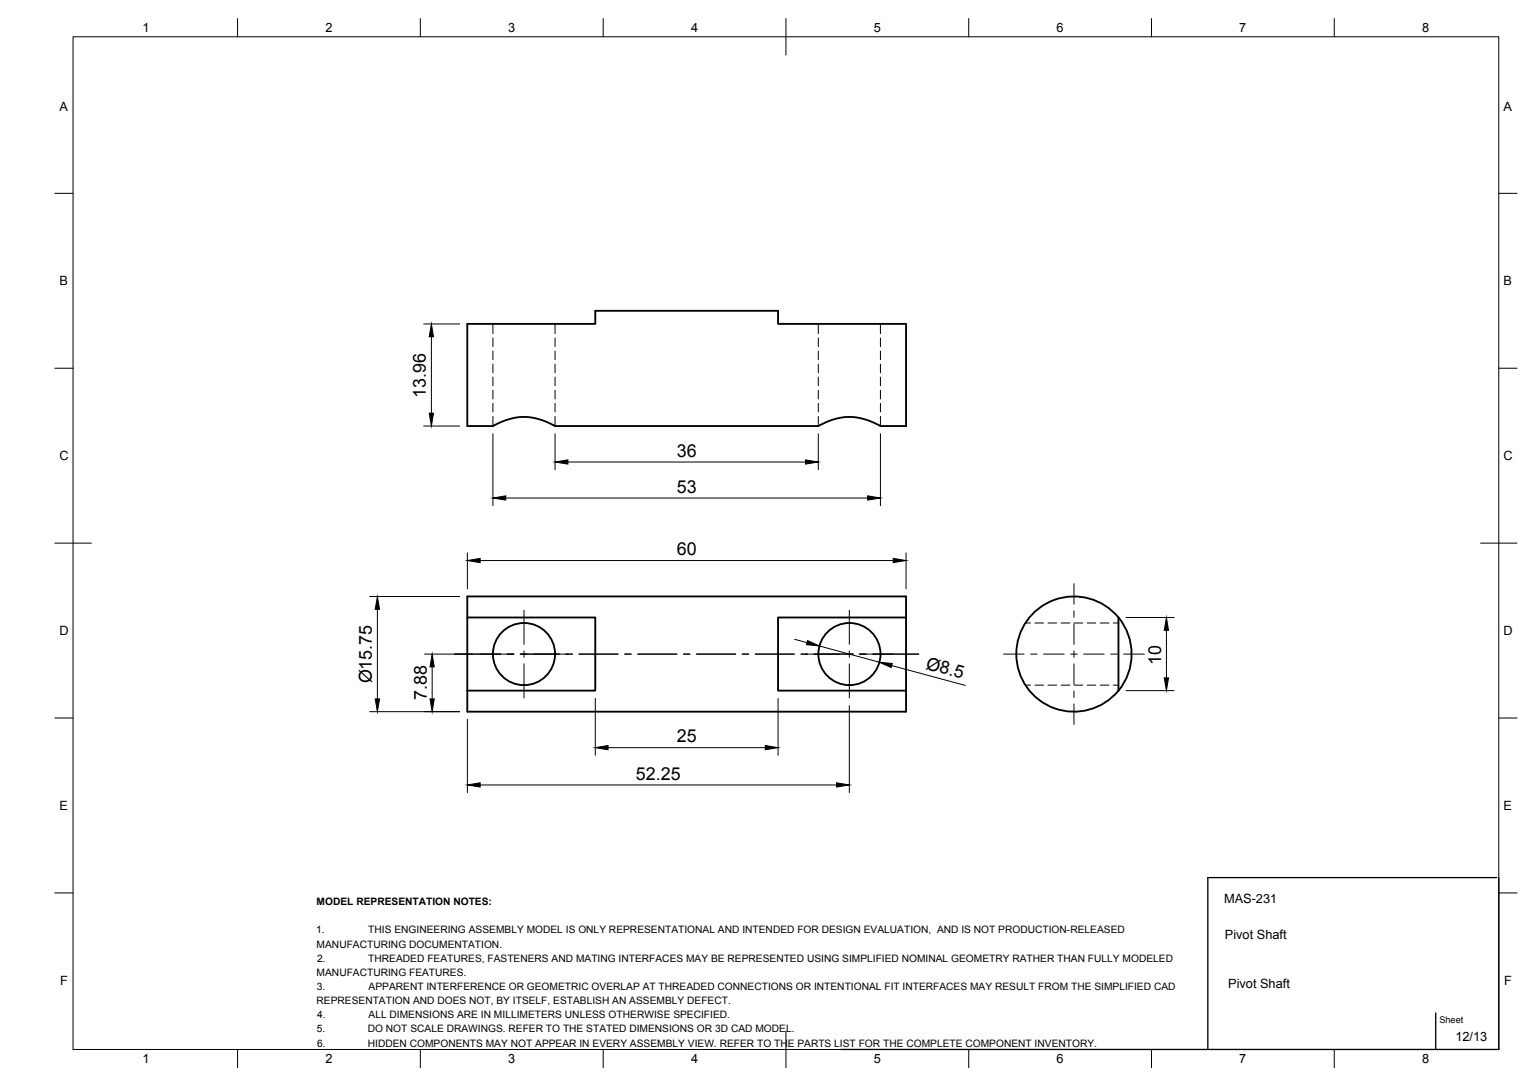
ISO-10303-21;
HEADER;
FILE_DESCRIPTION (('STEP AP214'),
    '1' );
FILE_NAME ( 'Pivot Shaft.step', '2026-10-04T02:08:54', ( '' ), ( '' ), 'STEP AP214', 'Unspecified', '' );
FILE_SCHEMA (( 'AUTOMOTIVE_DESIGN' ));
ENDSEC;
DATA;
#94=LINE ( 'NONE', #8474, #24641 ) ;
#163=CARTESIAN_POINT ( 'NONE',  ( 0.000000000000000000, 0.000000000000000000, 1.181102362204724310 ) ) ;
#167=FACE_BOUND ( 'NONE', #12224, .T. ) ;
#448=CARTESIAN_POINT ( 'NONE',  ( -0.3100393700787401619, -2.714815113292586694E-26, 1.043307086614172707 ) ) ;
#641=CARTESIAN_POINT ( 'NONE',  ( -0.3094175599200251203, 0.02245875686878780197, -0.7098059324661201153 ) ) ;
#676=CARTESIAN_POINT ( 'NONE',  ( -0.2802144182493691016, 0.1328525842424023995, 0.9782784368059546098 ) ) ;
#685=CARTESIAN_POINT ( 'NONE',  ( 0.2395294000716133853, 0.1968503937007874127, -1.181102362204724310 ) ) ;
#708=B_SPLINE_CURVE_WITH_KNOTS ( 'NONE', 3,
 ( #28141, #32202, #2466, #28627, #9914, #21640, #28865, #17093, #7013, #18040, #32685, #28374, #6538, #32454, #24524, #2926, #25235, #7260, #47275, #6296, #31966, #42943, #39824, #46788, #14454, #29112, #43665, #35327, #13976, #46551, #21152, #25494, #20919, #10153, #47031, #17804, #35559, #10873 ),
 .UNSPECIFIED., .F., .F.,
 ( 4, 2, 2, 2, 2, 2, 2, 2, 2, 2, 2, 2, 2, 2, 2, 2, 2, 2, 4 ),
 ( 0.000000000000000000, 0.0008476847199669468704, 0.001695369439933893741, 0.002543054159900840286, 0.003390738879867787482, 0.004238423599834733810, 0.005086108319801680572, 0.005933793039768628201, 0.006781477759735574963, 0.007205320119719049211, 0.007629162479702521725, 0.008476847199669457211, 0.009324531919636393565, 0.01017221663960332992, 0.01101990135957026627, 0.01186758607953720263, 0.01229142843952067167, 0.01271527079950414071, 0.01356295551947107707 ),
 .UNSPECIFIED. ) ;
#738=ADVANCED_FACE ( 'NONE', ( #36391 ), #37067, .F. ) ;
#834=VECTOR ( 'NONE', #5877, 39.37007874015748143 ) ;
#862=CARTESIAN_POINT ( 'NONE',  ( 0.2395294000716133853, 0.000000000000000000, 0.8759842519685039353 ) ) ;
#983=ORIENTED_EDGE ( 'NONE', *, *, #25046, .T. ) ;
#1196=AXIS2_PLACEMENT_3D ( 'NONE', #37509, #40374, #15249 ) ;
#1391=ORIENTED_EDGE ( 'NONE', *, *, #22168, .T. ) ;
#1402=DIRECTION ( 'NONE',  ( -1.000000000000000000, 0.000000000000000000, 0.000000000000000000 ) ) ;
#1442=CARTESIAN_POINT ( 'NONE',  ( -0.3100393700787401619, -2.714815113292586694E-26, 1.043307086614172707 ) ) ;
#1445=ADVANCED_FACE ( 'NONE', ( #167, #29705 ), #40878, .F. ) ;
#1497=CARTESIAN_POINT ( 'NONE',  ( 0.000000000000000000, 0.000000000000000000, -0.4921259842519685179 ) ) ;
#1651=VERTEX_POINT ( 'NONE', #38262 ) ;
#1728=CARTESIAN_POINT ( 'NONE',  ( -0.2984771744461587883, -0.08441368980803264088, 1.020863600671442217 ) ) ;
#1893=VERTEX_POINT ( 'NONE', #8023 ) ;
#2183=LINE ( 'NONE', #28090, #23824 ) ;
#2229=CARTESIAN_POINT ( 'NONE',  ( 0.2395294000716134131, 3.423225304703229610E-16, -0.7086614173228350522 ) ) ;
#2328=VERTEX_POINT ( 'NONE', #25156 ) ;
#2358=AXIS2_PLACEMENT_3D ( 'NONE', #3227, #47084, #17858 ) ;
#2433=EDGE_CURVE ( 'NONE', #33511, #19692, #3856, .T. ) ;
#2466=CARTESIAN_POINT ( 'NONE',  ( -0.3094241246319156535, -0.02236840013889242890, -1.042174736855756789 ) ) ;
#2926=CARTESIAN_POINT ( 'NONE',  ( -0.2617501178043720178, -0.1661865978653772336, -0.8983733778024277639 ) ) ;
#3106=FACE_OUTER_BOUND ( 'NONE', #33784, .T. ) ;
#3227=CARTESIAN_POINT ( 'NONE',  ( 0.2395294000716134131, 0.000000000000000000, 0.8759842519685039353 ) ) ;
#3244=ORIENTED_EDGE ( 'NONE', *, *, #38358, .T. ) ;
#3264=CARTESIAN_POINT ( 'NONE',  ( 0.000000000000000000, 0.000000000000000000, -1.181102362204724310 ) ) ;
#3298=DIRECTION ( 'NONE',  ( 0.000000000000000000, 0.000000000000000000, -1.000000000000000000 ) ) ;
#3333=ORIENTED_EDGE ( 'NONE', *, *, #7261, .F. ) ;
#3453=LINE ( 'NONE', #20944, #35658 ) ;
#3579=CARTESIAN_POINT ( 'NONE',  ( -0.3100393700787401619, 0.000000000000000000, 1.181102362204724310 ) ) ;
#3714=CARTESIAN_POINT ( 'NONE',  ( 0.2395294000716133853, 3.218313930830148909E-16, -0.8759842519685039353 ) ) ;
#3769=DIRECTION ( 'NONE',  ( 1.000000000000000000, -0.000000000000000000, -0.000000000000000000 ) ) ;
#3813=FACE_BOUND ( 'NONE', #38772, .T. ) ;
#3816=CARTESIAN_POINT ( 'NONE',  ( -0.3009843105729483326, 0.07510662309419850746, 1.025909792018103728 ) ) ;
#3856=B_SPLINE_CURVE_WITH_KNOTS ( 'NONE', 3,
 ( #448, #33557, #25878, #36658, #26118, #3816, #8360, #22985, #18436, #22034, #676, #11745, #14616, #15102, #7884, #11034, #33088, #37121, #7645, #22260, #36895, #4050, #18666, #4269, #15330, #29984, #8595, #30445, #41396, #42112, #44999, #34970, #38077, #23475 ),
 .UNSPECIFIED., .F., .F.,
 ( 4, 2, 2, 2, 2, 2, 2, 2, 2, 2, 2, 2, 2, 2, 2, 2, 4 ),
 ( 0.01356295551947108401, 0.01440869495260772501, 0.01525443438574436775, 0.01610017381888101048, 0.01694591325201764975, 0.01779165268515429249, 0.01863739211829093523, 0.01948313155142757797, 0.02032887098456421723, 0.02117461041770085997, 0.02202034985083749924, 0.02286608928397414198, 0.02371182871711078471, 0.02455756815024742745, 0.02540330758338407019, 0.02624904701652071293, 0.02709478644965735220 ),
 .UNSPECIFIED. ) ;
#3999=DIRECTION ( 'NONE',  ( 0.000000000000000000, -1.000000000000000000, 0.000000000000000000 ) ) ;
#4015=CARTESIAN_POINT ( 'NONE',  ( -0.2801604161619158928, 0.1329643277078512986, -0.9781273115788398087 ) ) ;
#4050=CARTESIAN_POINT ( 'NONE',  ( -0.2713217623817691382, 0.1501096695199154452, 0.8012500425422474093 ) ) ;
#4082=ORIENTED_EDGE ( 'NONE', *, *, #37554, .T. ) ;
#4221=DIRECTION ( 'NONE',  ( 0.000000000000000000, 0.000000000000000000, -1.000000000000000000 ) ) ;
#4253=LINE ( 'NONE', #3579, #24031 ) ;
#4269=CARTESIAN_POINT ( 'NONE',  ( -0.2801604161619160038, 0.1329643277078509933, 0.7738411923581678398 ) ) ;
#4359=CARTESIAN_POINT ( 'NONE',  ( -0.2801779484932495623, -0.1329283866310996265, 0.7737913416150018486 ) ) ;
#4376=DIRECTION ( 'NONE',  ( 1.000000000000000000, -0.000000000000000000, -0.000000000000000000 ) ) ;
#4465=CARTESIAN_POINT ( 'NONE',  ( -0.2664436179446793562, 0.1586070934160171142, -0.9304076372001184314 ) ) ;
#4696=ORIENTED_EDGE ( 'NONE', *, *, #24787, .F. ) ;
#4707=DIRECTION ( 'NONE',  ( -0.000000000000000000, 0.000000000000000000, 1.000000000000000000 ) ) ;
#4845=CARTESIAN_POINT ( 'NONE',  ( -0.2610212580023194007, -0.1673090378115814347, 0.8646000909489542918 ) ) ;
#4961=CARTESIAN_POINT ( 'NONE',  ( -0.3100393700787401619, 0.000000000000000000, 1.181102362204724310 ) ) ;
#4985=CARTESIAN_POINT ( 'NONE',  ( 0.2395294000716133853, 3.218313930830148909E-16, -1.043307086614172707 ) ) ;
#5087=CARTESIAN_POINT ( 'NONE',  ( -0.3076751137723113261, -0.03860885780051057786, 1.038887198594754979 ) ) ;
#5445=CIRCLE ( 'NONE', #2358, 0.1673228346456689108 ) ;
#5565=CARTESIAN_POINT ( 'NONE',  ( -0.2644880271752204637, -0.1617936740470132251, 0.8319153819575217934 ) ) ;
#5704=VECTOR ( 'NONE', #32125, 39.37007874015748143 ) ;
#5761=( LENGTH_UNIT ( ) NAMED_UNIT ( * ) SI_UNIT ( $, .METRE. ) ) ;
#5781=CIRCLE ( 'NONE', #7335, 0.3100393700787401619 ) ;
#5860=ORIENTED_EDGE ( 'NONE', *, *, #13221, .F. ) ;
#5877=DIRECTION ( 'NONE',  ( -0.000000000000000000, -0.000000000000000000, -1.000000000000000000 ) ) ;
#5938=PRODUCT_DEFINITION_SHAPE ( 'NONE', 'NONE',  #33920 ) ;
#6034=EDGE_CURVE ( 'NONE', #15025, #33889, #41592, .T. ) ;
#6150=ADVANCED_FACE ( 'NONE', ( #36097 ), #26746, .T. ) ;
#6209=DIRECTION ( 'NONE',  ( 0.000000000000000000, 0.000000000000000000, -1.000000000000000000 ) ) ;
#6296=CARTESIAN_POINT ( 'NONE',  ( -0.2618967166504349575, -0.1659366058165109570, -0.8537719073895772004 ) ) ;
#6351=( NAMED_UNIT ( * ) PLANE_ANGLE_UNIT ( ) SI_UNIT ( $, .RADIAN. ) ) ;
#6494=DIRECTION ( 'NONE',  ( 0.000000000000000000, 0.000000000000000000, -1.000000000000000000 ) ) ;
#6538=CARTESIAN_POINT ( 'NONE',  ( -0.2713482210566314223, -0.1500601874062439112, -0.9507959855109898717 ) ) ;
#6942=CARTESIAN_POINT ( 'NONE',  ( 0.2395294000716133853, 0.000000000000000000, 0.8759842519685039353 ) ) ;
#7013=CARTESIAN_POINT ( 'NONE',  ( -0.2896304277639956681, -0.1109299681405381544, -1.001705941724043258 ) ) ;
#7184=ORIENTED_EDGE ( 'NONE', *, *, #17160, .T. ) ;
#7260=CARTESIAN_POINT ( 'NONE',  ( -0.2610081115717082234, -0.1673295453843248459, -0.8705991056603238354 ) ) ;
#7261=EDGE_CURVE ( 'NONE', #27285, #2328, #3453, .T. ) ;
#7264=AXIS2_PLACEMENT_3D ( 'NONE', #44630, #4376, #12327 ) ;
#7283=ORIENTED_EDGE ( 'NONE', *, *, #41575, .F. ) ;
#7286=DIRECTION ( 'NONE',  ( -0.000000000000000000, -0.000000000000000000, 1.000000000000000000 ) ) ;
#7314=( NAMED_UNIT ( * ) SI_UNIT ( $, .STERADIAN. ) SOLID_ANGLE_UNIT ( ) ) ;
#7335=AXIS2_PLACEMENT_3D ( 'NONE', #19833, #27300, #34463 ) ;
#7380=DIRECTION ( 'NONE',  ( 0.000000000000000000, 0.000000000000000000, -1.000000000000000000 ) ) ;
#7412=PLANE ( 'NONE',  #17888 ) ;
#7612=CARTESIAN_POINT ( 'NONE',  ( -0.2644617891023671730, 0.1618364700813167412, -0.9199053124863334485 ) ) ;
#7645=CARTESIAN_POINT ( 'NONE',  ( -0.2617290863461586570, 0.1662196327273371133, 0.8538226567781561638 ) ) ;
#7733=STYLED_ITEM ( 'NONE', ( #47336 ), #20411 ) ;
#7830=ORIENTED_EDGE ( 'NONE', *, *, #45870, .F. ) ;
#7884=CARTESIAN_POINT ( 'NONE',  ( -0.2645270498714851759, 0.1617305326345081506, 0.9203172363904412734 ) ) ;
#8023=CARTESIAN_POINT ( 'NONE',  ( 0.2395294000716133853, 0.1968503937007874127, 1.181102362204724310 ) ) ;
#8208=CARTESIAN_POINT ( 'NONE',  ( -0.2984316586355670875, -0.08457185433607530833, 0.7311987702743616424 ) ) ;
#8332=EDGE_LOOP ( 'NONE', ( #7283, #23510, #23532, #30825 ) ) ;
#8359=AXIS2_PLACEMENT_3D ( 'NONE', #862, #3769, #4221 ) ;
#8360=CARTESIAN_POINT ( 'NONE',  ( -0.2984108399384687305, 0.08463831125274398626, 1.020725522217017955 ) ) ;
#8474=CARTESIAN_POINT ( 'NONE',  ( 0.2395294000716133853, 0.1968503937007874127, -0.4921259842519685179 ) ) ;
#8498=EDGE_CURVE ( 'NONE', #42416, #16713, #45273, .T. ) ;
#8595=CARTESIAN_POINT ( 'NONE',  ( -0.2926984831716178959, 0.1026671379286196728, 0.7434188456247464716 ) ) ;
#8721=ORIENTED_EDGE ( 'NONE', *, *, #11537, .T. ) ;
#8762=CLOSED_SHELL ( 'NONE', ( #26435, #738, #32463, #29801, #29703, #38357, #37221, #36225, #1445, #6150, #37716, #20453 ) ) ;
#8798=DIRECTION ( 'NONE',  ( 0.000000000000000000, 1.000000000000000000, 0.000000000000000000 ) ) ;
#8930=CARTESIAN_POINT ( 'NONE',  ( -0.2644738720849207914, -0.1618167320693824351, 0.9199706799918920819 ) ) ;
#9023=DIMENSIONAL_EXPONENTS ( 1.000000000000000000, 0.000000000000000000, 0.000000000000000000, 0.000000000000000000, 0.000000000000000000, 0.000000000000000000, 0.000000000000000000 ) ;
#9122=( CONVERSION_BASED_UNIT ( 'INCH', #27605 ) LENGTH_UNIT ( ) NAMED_UNIT ( #20041 ) ) ;
#9166=CARTESIAN_POINT ( 'NONE',  ( -0.2834275672170630811, -0.1259372798753287670, 0.9866696916589494659 ) ) ;
#9181=PLANE ( 'NONE',  #23201 ) ;
#9239=AXIS2_PLACEMENT_3D ( 'NONE', #19213, #30507, #22810 ) ;
#9246=AXIS2_PLACEMENT_3D ( 'NONE', #3714, #10688, #21205 ) ;
#9284=CARTESIAN_POINT ( 'NONE',  ( -0.3100393700787401619, 3.218313930830148909E-16, -1.043307086614172707 ) ) ;
#9328=ORIENTED_EDGE ( 'NONE', *, *, #2433, .F. ) ;
#9410=CARTESIAN_POINT ( 'NONE',  ( -0.3100393700787403284, -0.01116717051762142893, 1.043307086614172929 ) ) ;
#9577=ORIENTED_EDGE ( 'NONE', *, *, #41668, .F. ) ;
#9664=DIRECTION ( 'NONE',  ( -1.000000000000000000, 0.000000000000000000, -0.000000000000000000 ) ) ;
#9829=ORIENTED_EDGE ( 'NONE', *, *, #32167, .T. ) ;
#9914=CARTESIAN_POINT ( 'NONE',  ( -0.3053278657842540267, -0.05482723079889029877, -1.034448866034457293 ) ) ;
#9995=DIRECTION ( 'NONE',  ( -1.000000000000000000, 0.000000000000000000, 0.000000000000000000 ) ) ;
#9998=DIRECTION ( 'NONE',  ( -1.000000000000000000, 0.000000000000000000, 0.000000000000000000 ) ) ;
#10039=COLOUR_RGB ( '', 0.08235294, 0.09019608, 0.10196078) ;
#10059=AXIS2_PLACEMENT_3D ( 'NONE', #33792, #24392, #27791 ) ;
#10153=CARTESIAN_POINT ( 'NONE',  ( -0.3069380822740675474, -0.04406989549021587960, -0.7144743529967967355 ) ) ;
#10559=VECTOR ( 'NONE', #43712, 39.37007874015748143 ) ;
#10688=DIRECTION ( 'NONE',  ( 1.000000000000000000, -0.000000000000000000, -0.000000000000000000 ) ) ;
#10732=VECTOR ( 'NONE', #3999, 39.37007874015748143 ) ;
#10774=CARTESIAN_POINT ( 'NONE',  ( -0.3010001048904012433, 0.07502508536398735939, -1.025940429181291913 ) ) ;
#10835=DIRECTION ( 'NONE',  ( 1.000000000000000000, 0.000000000000000000, 0.000000000000000000 ) ) ;
#10873=CARTESIAN_POINT ( 'NONE',  ( -0.3100393700787401619, -2.714815113292586694E-26, -0.7086614173228351632 ) ) ;
#10880=DIRECTION ( 'NONE',  ( 0.000000000000000000, 0.000000000000000000, -1.000000000000000000 ) ) ;
#10897=CARTESIAN_POINT ( 'NONE',  ( -0.2927220607601821456, -0.1026043301529240143, 0.7433660568023925386 ) ) ;
#11034=CARTESIAN_POINT ( 'NONE',  ( -0.2617458567146320192, 0.1661939583519094210, 0.8983839595853735371 ) ) ;
#11236=CARTESIAN_POINT ( 'NONE',  ( -0.2645270498714851204, 0.1617305326345083449, -0.8316512675465659310 ) ) ;
#11359=CARTESIAN_POINT ( 'NONE',  ( -0.3094241246319155980, -0.02236840013889274115, 0.7097937670812509703 ) ) ;
#11367=SHAPE_DEFINITION_REPRESENTATION ( #5938, #19102 ) ;
#11506=CARTESIAN_POINT ( 'NONE',  ( 0.3100393700787401619, 0.000000000000000000, 1.181102362204724310 ) ) ;
#11537=EDGE_CURVE ( 'NONE', #1651, #19863, #29118, .T. ) ;
#11587=AXIS2_PLACEMENT_3D ( 'NONE', #34729, #41865, #34475 ) ;
#11593=CARTESIAN_POINT ( 'NONE',  ( -0.3053278657842537491, -0.05482723079889069429, 0.7175196379025509108 ) ) ;
#11616=AXIS2_PLACEMENT_3D ( 'NONE', #16375, #20181, #17531 ) ;
#11693=LINE ( 'NONE', #22213, #10732 ) ;
#11708=CARTESIAN_POINT ( 'NONE',  ( -0.3009843105729483326, 0.07510662309419861848, -0.7260587119189039207 ) ) ;
#11745=CARTESIAN_POINT ( 'NONE',  ( -0.2741699206993517546, 0.1449164722121958904, 0.9603235990907990072 ) ) ;
#11935=CARTESIAN_POINT ( 'NONE',  ( 0.2395294000716133853, 0.1968503937007874127, 0.4921259842519685179 ) ) ;
#11947=CARTESIAN_POINT ( 'NONE',  ( -0.3070313825494068727, 0.04447134000132169085, -1.037676521114162531 ) ) ;
#12224=EDGE_LOOP ( 'NONE', ( #15611, #33162 ) ) ;
#12327=DIRECTION ( 'NONE',  ( 0.000000000000000000, 0.000000000000000000, -1.000000000000000000 ) ) ;
#12341=CARTESIAN_POINT ( 'NONE',  ( 0.2395294000716133853, 0.1968503937007874127, 1.181102362204724310 ) ) ;
#12412=CARTESIAN_POINT ( 'NONE',  ( 0.2395294000716133853, 0.1968503937007874127, 0.4921259842519685179 ) ) ;
#12472=DIRECTION ( 'NONE',  ( 1.000000000000000000, 0.000000000000000000, 0.000000000000000000 ) ) ;
#12779=CARTESIAN_POINT ( 'NONE',  ( -0.2624241468390500209, -0.1651049555683128389, 0.9036955682336973439 ) ) ;
#12865=VECTOR ( 'NONE', #10880, 39.37007874015748143 ) ;
#12920=CARTESIAN_POINT ( 'NONE',  ( -0.3100393700787401619, 0.000000000000000000, 1.181102362204724310 ) ) ;
#13009=CARTESIAN_POINT ( 'NONE',  ( -0.2741778990008359451, -0.1449014624352428227, 0.9603494317905525435 ) ) ;
#13087=EDGE_CURVE ( 'NONE', #47237, #42416, #21013, .T. ) ;
#13221=EDGE_CURVE ( 'NONE', #18450, #33511, #42079, .T. ) ;
#13498=CARTESIAN_POINT ( 'NONE',  ( -0.3100393700787401619, 0.000000000000000000, 0.7086614173228351632 ) ) ;
#13509=ORIENTED_EDGE ( 'NONE', *, *, #46510, .F. ) ;
#13549=CARTESIAN_POINT ( 'NONE',  ( 0.2395294000716134131, 3.218313930830148909E-16, -0.8759842519685039353 ) ) ;
#13869=CIRCLE ( 'NONE', #11587, 0.1673228346456689108 ) ;
#13899=DIRECTION ( 'NONE',  ( -1.000000000000000000, 0.000000000000000000, 0.000000000000000000 ) ) ;
#13976=CARTESIAN_POINT ( 'NONE',  ( -0.2927617443614863313, -0.1024931984611133912, -0.7432784081755305916 ) ) ;
#14140=CIRCLE ( 'NONE', #40883, 0.1673228346456689108 ) ;
#14357=CARTESIAN_POINT ( 'NONE',  ( -0.2713217623817689717, 0.1501096695199156672, -0.9507184613947605722 ) ) ;
#14454=CARTESIAN_POINT ( 'NONE',  ( -0.2741778990008360561, -0.1449014624352426839, -0.7916190721464555491 ) ) ;
#14585=CARTESIAN_POINT ( 'NONE',  ( -0.2617290863461584904, 0.1662196327273373908, -0.8981458471588513737 ) ) ;
#14616=CARTESIAN_POINT ( 'NONE',  ( -0.2713383277233172297, 0.1500775187160213187, 0.9507557288134271811 ) ) ;
#14695=CARTESIAN_POINT ( 'NONE',  ( 0.3100393700787401619, 3.796887221765908018E-17, 1.181102362204724310 ) ) ;
#15025=VERTEX_POINT ( 'NONE', #37434 ) ;
#15087=DIRECTION ( 'NONE',  ( 0.000000000000000000, 0.000000000000000000, -1.000000000000000000 ) ) ;
#15102=CARTESIAN_POINT ( 'NONE',  ( -0.2665307357296562429, 0.1584585643853060888, 0.9308013911357060355 ) ) ;
#15110=FACE_OUTER_BOUND ( 'NONE', #18912, .T. ) ;
#15200=PRODUCT_CONTEXT ( 'NONE', #37994, 'mechanical' ) ;
#15249=DIRECTION ( 'NONE',  ( 1.000000000000000000, 0.000000000000000000, -0.000000000000000000 ) ) ;
#15294=CARTESIAN_POINT ( 'NONE',  ( -0.3070711847658871285, 0.04416910270118660359, -0.7142167645079522398 ) ) ;
#15330=CARTESIAN_POINT ( 'NONE',  ( -0.2833779466431470828, 0.1260493684579866713, 0.7654247733636371231 ) ) ;
#15444=FACE_OUTER_BOUND ( 'NONE', #31318, .T. ) ;
#15595=CIRCLE ( 'NONE', #42341, 0.3100393700787401619 ) ;
#15611=ORIENTED_EDGE ( 'NONE', *, *, #20592, .F. ) ;
#15670=CARTESIAN_POINT ( 'NONE',  ( -0.2611872605799124836, -0.1670510767787602990, 0.8870424230945959110 ) ) ;
#15902=ORIENTED_EDGE ( 'NONE', *, *, #30363, .T. ) ;
#16004=LINE ( 'NONE', #12412, #45142 ) ;
#16250=CARTESIAN_POINT ( 'NONE',  ( -0.3100393700787401619, 0.01127274112884939748, -1.043307086614172263 ) ) ;
#16375=CARTESIAN_POINT ( 'NONE',  ( 0.000000000000000000, 0.000000000000000000, -0.4921259842519685179 ) ) ;
#16466=VECTOR ( 'NONE', #23016, 39.37007874015748143 ) ;
#16479=EDGE_LOOP ( 'NONE', ( #42150, #27237, #15902 ) ) ;
#16713=VERTEX_POINT ( 'NONE', #32228 ) ;
#16906=CARTESIAN_POINT ( 'NONE',  ( 0.2395294000716133853, 0.1968503937007874127, 0.4921259842519685179 ) ) ;
#16951=CARTESIAN_POINT ( 'NONE',  ( 0.000000000000000000, 0.000000000000000000, -0.4921259842519685179 ) ) ;
#17093=CARTESIAN_POINT ( 'NONE',  ( -0.2927220607601823121, -0.1026043301529236951, -1.008602447134615776 ) ) ;
#17160=EDGE_CURVE ( 'NONE', #42416, #47237, #708, .T. ) ;
#17224=UNCERTAINTY_MEASURE_WITH_UNIT (LENGTH_MEASURE( 1.000000000000000082E-05 ), #18094, 'distance_accuracy_value', 'NONE') ;
#17388=ORIENTED_EDGE ( 'NONE', *, *, #21147, .F. ) ;
#17521=CARTESIAN_POINT ( 'NONE',  ( 0.2395294000716134131, 3.218313930830148909E-16, -0.8759842519685039353 ) ) ;
#17531=DIRECTION ( 'NONE',  ( -1.000000000000000000, 0.000000000000000000, 0.000000000000000000 ) ) ;
#17576=ORIENTED_EDGE ( 'NONE', *, *, #6034, .T. ) ;
#17715=DIRECTION ( 'NONE',  ( 0.000000000000000000, 0.000000000000000000, 1.000000000000000000 ) ) ;
#17804=CARTESIAN_POINT ( 'NONE',  ( -0.3094378032379023757, -0.02221465895966925203, -0.7097682129517437488 ) ) ;
#17858=DIRECTION ( 'NONE',  ( 0.000000000000000000, 0.000000000000000000, -1.000000000000000000 ) ) ;
#17888=AXIS2_PLACEMENT_3D ( 'NONE', #40222, #13899, #21313 ) ;
#18040=CARTESIAN_POINT ( 'NONE',  ( -0.2833820772873882343, -0.1260390447071882414, -0.9865535077132553399 ) ) ;
#18056=CIRCLE ( 'NONE', #24198, 0.3100393700787401619 ) ;
#18094=( CONVERSION_BASED_UNIT ( 'INCH', #24580 ) LENGTH_UNIT ( ) NAMED_UNIT ( #9023 ) ) ;
#18298=EDGE_CURVE ( 'NONE', #32711, #37242, #13869, .T. ) ;
#18432=CARTESIAN_POINT ( 'NONE',  ( 0.2395294000716134131, 0.000000000000000000, 0.7086614173228350522 ) ) ;
#18436=CARTESIAN_POINT ( 'NONE',  ( -0.2896200801440090289, 0.1109568837733816149, 1.001682203372160851 ) ) ;
#18450=VERTEX_POINT ( 'NONE', #12920 ) ;
#18452=VERTEX_POINT ( 'NONE', #20784 ) ;
#18522=EDGE_LOOP ( 'NONE', ( #37211, #45478, #25610 ) ) ;
#18634=CARTESIAN_POINT ( 'NONE',  ( -0.2833779466431469163, 0.1260493684579870322, -0.9865437305733709694 ) ) ;
#18666=CARTESIAN_POINT ( 'NONE',  ( -0.2741498948998221663, 0.1449524278970008850, 0.7917137902625999146 ) ) ;
#18754=ORIENTED_EDGE ( 'NONE', *, *, #43762, .T. ) ;
#18761=CARTESIAN_POINT ( 'NONE',  ( -0.3100393700787401619, 0.000000000000000000, 0.7086614173228351632 ) ) ;
#18878=VERTEX_POINT ( 'NONE', #16906 ) ;
#18912=EDGE_LOOP ( 'NONE', ( #46093, #4696, #36297, #24814, #41189, #21892, #983, #28641, #38448, #20562, #7830, #32610 ) ) ;
#18991=ORIENTED_EDGE ( 'NONE', *, *, #30363, .F. ) ;
#19094=ORIENTED_EDGE ( 'NONE', *, *, #30673, .F. ) ;
#19102=SHAPE_REPRESENTATION ( 'Pivot Shaft', ( #20860 ), #43813 ) ;
#19128=CYLINDRICAL_SURFACE ( 'NONE', #10059, 0.3100393700787401619 ) ;
#19213=CARTESIAN_POINT ( 'NONE',  ( 0.000000000000000000, 0.000000000000000000, 0.4921259842519685179 ) ) ;
#19588=DIRECTION ( 'NONE',  ( 0.000000000000000000, 0.000000000000000000, -1.000000000000000000 ) ) ;
#19692=VERTEX_POINT ( 'NONE', #13498 ) ;
#19709=CARTESIAN_POINT ( 'NONE',  ( -0.3069380822740674364, -0.04406989549021581021, 1.037494150940211357 ) ) ;
#19822=CARTESIAN_POINT ( 'NONE',  ( -0.3094147346904633222, 0.02254976514608475827, -1.042157649583289158 ) ) ;
#19833=CARTESIAN_POINT ( 'NONE',  ( 0.000000000000000000, 0.000000000000000000, -1.181102362204724310 ) ) ;
#19863=VERTEX_POINT ( 'NONE', #38551 ) ;
#19889=ORIENTED_EDGE ( 'NONE', *, *, #21147, .T. ) ;
#20041=DIMENSIONAL_EXPONENTS ( 1.000000000000000000, 0.000000000000000000, 0.000000000000000000, 0.000000000000000000, 0.000000000000000000, 0.000000000000000000, 0.000000000000000000 ) ;
#20176=CARTESIAN_POINT ( 'NONE',  ( -0.2665235116888309275, -0.1584712422872024407, 0.8211962908093238811 ) ) ;
#20181=DIRECTION ( 'NONE',  ( 0.000000000000000000, 0.000000000000000000, -1.000000000000000000 ) ) ;
#20246=CARTESIAN_POINT ( 'NONE',  ( 0.2395294000716133853, -0.1968503937007874127, -0.4921259842519685179 ) ) ;
#20411=MANIFOLD_SOLID_BREP ( 'Pivot Shaft', #8762 ) ;
#20453=ADVANCED_FACE ( 'NONE', ( #43722 ), #36554, .F. ) ;
#20562=ORIENTED_EDGE ( 'NONE', *, *, #43163, .F. ) ;
#20592=EDGE_CURVE ( 'NONE', #37242, #32711, #5445, .T. ) ;
#20641=DIRECTION ( 'NONE',  ( 1.000000000000000000, -0.000000000000000000, -0.000000000000000000 ) ) ;
#20784=CARTESIAN_POINT ( 'NONE',  ( 0.2395294000716134131, 3.218313930830148909E-16, -1.043307086614172929 ) ) ;
#20838=DIRECTION ( 'NONE',  ( -1.000000000000000000, 0.000000000000000000, 0.000000000000000000 ) ) ;
#20860=AXIS2_PLACEMENT_3D ( 'NONE', #25692, #32652, #10835 ) ;
#20919=CARTESIAN_POINT ( 'NONE',  ( -0.3052312982475722247, -0.05465342266228452595, -0.7177420118880897260 ) ) ;
#20944=CARTESIAN_POINT ( 'NONE',  ( 0.2395294000716133853, -0.1968503937007874127, 0.4921259842519685179 ) ) ;
#20959=DIRECTION ( 'NONE',  ( 0.000000000000000000, 0.000000000000000000, -1.000000000000000000 ) ) ;
#21013=B_SPLINE_CURVE_WITH_KNOTS ( 'NONE', 3,
 ( #47411, #33525, #641, #15294, #36628, #11708, #26333, #39961, #29491, #32586, #22227, #44035, #40894, #37316, #11236, #21778, #25847, #40429, #14585, #7612, #4465, #14357, #36860, #4015, #18634, #29259, #33294, #29005, #10774, #37561, #11947, #19822, #16250, #9284 ),
 .UNSPECIFIED., .F., .F.,
 ( 4, 2, 2, 2, 2, 2, 2, 2, 2, 2, 2, 2, 2, 2, 2, 2, 4 ),
 ( 0.01356295551947107707, 0.01440869495260771981, 0.01525443438574436081, 0.01610017381888100355, 0.01694591325201764628, 0.01779165268515428555, 0.01863739211829092829, 0.01948313155142757103, 0.02032887098456421376, 0.02117461041770085650, 0.02202034985083749924, 0.02286608928397414198, 0.02371182871711078471, 0.02455756815024742745, 0.02540330758338407019, 0.02624904701652071293, 0.02709478644965735220 ),
 .UNSPECIFIED. ) ;
#21077=FACE_OUTER_BOUND ( 'NONE', #39620, .T. ) ;
#21082=LINE ( 'NONE', #12341, #5704 ) ;
#21147=EDGE_CURVE ( 'NONE', #19692, #37242, #2183, .T. ) ;
#21152=CARTESIAN_POINT ( 'NONE',  ( -0.3010365421720465617, -0.07487990393731468186, -0.7259551242400892335 ) ) ;
#21205=DIRECTION ( 'NONE',  ( 0.000000000000000000, 0.000000000000000000, -1.000000000000000000 ) ) ;
#21313=DIRECTION ( 'NONE',  ( 0.000000000000000000, 0.000000000000000000, 1.000000000000000000 ) ) ;
#21432=LINE ( 'NONE', #43232, #10559 ) ;
#21640=CARTESIAN_POINT ( 'NONE',  ( -0.3010010101267349136, -0.07503014570242684533, -1.025942700826908638 ) ) ;
#21778=CARTESIAN_POINT ( 'NONE',  ( -0.2617458567146319082, 0.1661939583519097263, -0.8535845443516340003 ) ) ;
#21892=ORIENTED_EDGE ( 'NONE', *, *, #47187, .F. ) ;
#22034=CARTESIAN_POINT ( 'NONE',  ( -0.2833714012347087752, 0.1260629598319807643, 0.9865262584736159690 ) ) ;
#22168=EDGE_CURVE ( 'NONE', #33889, #29837, #94, .T. ) ;
#22213=CARTESIAN_POINT ( 'NONE',  ( 0.2395294000716133853, 0.1968503937007874127, 0.4921259842519685179 ) ) ;
#22227=CARTESIAN_POINT ( 'NONE',  ( -0.2802144182493689351, 0.1328525842424026215, -0.7736900671310529276 ) ) ;
#22253=ORIENTED_EDGE ( 'NONE', *, *, #2433, .T. ) ;
#22260=CARTESIAN_POINT ( 'NONE',  ( -0.2644617891023673395, 0.1618364700813163526, 0.8320631914506742000 ) ) ;
#22539=ORIENTED_EDGE ( 'NONE', *, *, #6034, .F. ) ;
#22574=CIRCLE ( 'NONE', #34071, 0.3100393700787401619 ) ;
#22600=CARTESIAN_POINT ( 'NONE',  ( -0.2896304277639954461, -0.1109299681405384735, 0.7502625622129650562 ) ) ;
#22810=DIRECTION ( 'NONE',  ( 1.000000000000000000, 0.000000000000000000, 0.000000000000000000 ) ) ;
#22937=DIRECTION ( 'NONE',  ( -1.000000000000000000, 0.000000000000000000, -0.000000000000000000 ) ) ;
#22985=CARTESIAN_POINT ( 'NONE',  ( -0.2927386332256519674, 0.1025512834716171690, 1.008637609646301447 ) ) ;
#23016=DIRECTION ( 'NONE',  ( 0.000000000000000000, 0.000000000000000000, -1.000000000000000000 ) ) ;
#23201=AXIS2_PLACEMENT_3D ( 'NONE', #1497, #42459, #9664 ) ;
#23311=LINE ( 'NONE', #33884, #27164 ) ;
#23426=ORIENTED_EDGE ( 'NONE', *, *, #8498, .F. ) ;
#23475=CARTESIAN_POINT ( 'NONE',  ( -0.3100393700787401619, 0.000000000000000000, 0.7086614173228351632 ) ) ;
#23478=ORIENTED_EDGE ( 'NONE', *, *, #32167, .F. ) ;
#23510=ORIENTED_EDGE ( 'NONE', *, *, #13087, .T. ) ;
#23532=ORIENTED_EDGE ( 'NONE', *, *, #25281, .T. ) ;
#23554=CARTESIAN_POINT ( 'NONE',  ( -0.2713482210566312558, -0.1500601874062442720, 0.8011725184260182209 ) ) ;
#23659=VECTOR ( 'NONE', #19588, 39.37007874015748143 ) ;
#23663=CARTESIAN_POINT ( 'NONE',  ( 0.2395294000716133853, -0.1968503937007874127, -0.4921259842519685179 ) ) ;
#23773=VERTEX_POINT ( 'NONE', #2229 ) ;
#23783=( GEOMETRIC_REPRESENTATION_CONTEXT ( 3 ) GLOBAL_UNCERTAINTY_ASSIGNED_CONTEXT ( ( #17224 ) ) GLOBAL_UNIT_ASSIGNED_CONTEXT ( ( #18094, #6351, #7314 ) ) REPRESENTATION_CONTEXT ( 'NONE', 'WORKASPACE' ) ) ;
#23824=VECTOR ( 'NONE', #43136, 39.37007874015748143 ) ;
#23985=( NAMED_UNIT ( * ) SI_UNIT ( $, .STERADIAN. ) SOLID_ANGLE_UNIT ( ) ) ;
#24028=CARTESIAN_POINT ( 'NONE',  ( -0.3052312982475723357, -0.05465342266228453288, 1.034226492048918145 ) ) ;
#24031=VECTOR ( 'NONE', #15087, 39.37007874015748143 ) ;
#24198=AXIS2_PLACEMENT_3D ( 'NONE', #163, #3298, #24879 ) ;
#24222=SHAPE_REPRESENTATION_RELATIONSHIP ( 'NONE' , 'NONE' ,  #19102, #44979 ) ;
#24392=DIRECTION ( 'NONE',  ( 0.000000000000000000, 0.000000000000000000, -1.000000000000000000 ) ) ;
#24524=CARTESIAN_POINT ( 'NONE',  ( -0.2644880271752205192, -0.1617936740470128087, -0.9200531219794864102 ) ) ;
#24580=LENGTH_MEASURE_WITH_UNIT ( LENGTH_MEASURE( 0.02539999999999999897 ), #28679 ) ;
#24641=VECTOR ( 'NONE', #36548, 39.37007874015748143 ) ;
#24707=ORIENTED_EDGE ( 'NONE', *, *, #18298, .T. ) ;
#24783=EDGE_CURVE ( 'NONE', #2328, #18450, #28596, .T. ) ;
#24787=EDGE_CURVE ( 'NONE', #27285, #1651, #15595, .T. ) ;
#24811=FILL_AREA_STYLE ('',( #32740 ) ) ;
#24814=ORIENTED_EDGE ( 'NONE', *, *, #24783, .T. ) ;
#24879=DIRECTION ( 'NONE',  ( -1.000000000000000000, 0.000000000000000000, 0.000000000000000000 ) ) ;
#25046=EDGE_CURVE ( 'NONE', #19692, #47237, #4253, .T. ) ;
#25100=CARTESIAN_POINT ( 'NONE',  ( 0.2395294000716133853, -0.1968503937007874127, 0.4921259842519685179 ) ) ;
#25156=CARTESIAN_POINT ( 'NONE',  ( 0.2395294000716133853, -0.1968503937007874127, 1.181102362204724310 ) ) ;
#25235=CARTESIAN_POINT ( 'NONE',  ( -0.2610212580023196227, -0.1673090378115812127, -0.8873684129880539118 ) ) ;
#25281=EDGE_CURVE ( 'NONE', #42416, #18452, #34721, .T. ) ;
#25333=CIRCLE ( 'NONE', #43677, 0.1673228346456689108 ) ;
#25406=CIRCLE ( 'NONE', #11616, 0.3100393700787401619 ) ;
#25494=CARTESIAN_POINT ( 'NONE',  ( -0.3042596054108610559, -0.05980719604265496286, -0.7196201501354283492 ) ) ;
#25610=ORIENTED_EDGE ( 'NONE', *, *, #42114, .T. ) ;
#25692=CARTESIAN_POINT ( 'NONE',  ( 0.000000000000000000, 0.000000000000000000, 0.000000000000000000 ) ) ;
#25847=CARTESIAN_POINT ( 'NONE',  ( -0.2610236670165029249, 0.1673052798952545106, -0.8646194990212731080 ) ) ;
#25878=CARTESIAN_POINT ( 'NONE',  ( -0.3094175599200249538, 0.02245875686878769095, 1.042162571470887977 ) ) ;
#26118=CARTESIAN_POINT ( 'NONE',  ( -0.3053406547161471862, 0.05476901150469691559, 1.034474086880956989 ) ) ;
#26129=DIRECTION ( 'NONE',  ( 0.000000000000000000, 0.000000000000000000, -1.000000000000000000 ) ) ;
#26217=CARTESIAN_POINT ( 'NONE',  ( -0.3010010101267347471, -0.07503014570242728942, 0.7260258031100994547 ) ) ;
#26311=ORIENTED_EDGE ( 'NONE', *, *, #38358, .F. ) ;
#26333=CARTESIAN_POINT ( 'NONE',  ( -0.2984108399384686749, 0.08463831125274406952, -0.7312429817199896931 ) ) ;
#26435=ADVANCED_FACE ( 'NONE', ( #15444 ), #40800, .F. ) ;
#26690=CARTESIAN_POINT ( 'NONE',  ( -0.2617501178043717958, -0.1661865978653775666, 0.8535951261345801067 ) ) ;
#26701=CARTESIAN_POINT ( 'NONE',  ( 0.2395294000716133853, 2.049113738730801466E-17, 1.043307086614172707 ) ) ;
#26746=PLANE ( 'NONE',  #1196 ) ;
#26752=ORIENTED_EDGE ( 'NONE', *, *, #25281, .F. ) ;
#26839=CARTESIAN_POINT ( 'NONE',  ( 0.2395294000716133853, -0.1968503937007874127, -1.181102362204724310 ) ) ;
#27164=VECTOR ( 'NONE', #34341, 39.37007874015748143 ) ;
#27173=CARTESIAN_POINT ( 'NONE',  ( -0.2927617443614862758, -0.1024931984611135161, 1.008690095761477723 ) ) ;
#27237=ORIENTED_EDGE ( 'NONE', *, *, #31027, .T. ) ;
#27285=VERTEX_POINT ( 'NONE', #25100 ) ;
#27300=DIRECTION ( 'NONE',  ( 0.000000000000000000, 0.000000000000000000, -1.000000000000000000 ) ) ;
#27415=CARTESIAN_POINT ( 'NONE',  ( -0.2802233088437623976, -0.1328339237432898945, 0.9783027062435790677 ) ) ;
#27463=ORIENTED_EDGE ( 'NONE', *, *, #45870, .T. ) ;
#27605=LENGTH_MEASURE_WITH_UNIT ( LENGTH_MEASURE( 0.02539999999999999897 ), #5761 ) ;
#27791=DIRECTION ( 'NONE',  ( -1.000000000000000000, 0.000000000000000000, 0.000000000000000000 ) ) ;
#27818=ORIENTED_EDGE ( 'NONE', *, *, #43762, .F. ) ;
#28090=CARTESIAN_POINT ( 'NONE',  ( 0.2395294000716133853, 0.000000000000000000, 0.7086614173228351632 ) ) ;
#28141=CARTESIAN_POINT ( 'NONE',  ( -0.3100393700787401619, 3.218313930830148909E-16, -1.043307086614172707 ) ) ;
#28374=CARTESIAN_POINT ( 'NONE',  ( -0.2741503469832766160, -0.1449524958156367394, -0.9602583337237132755 ) ) ;
#28432=SURFACE_STYLE_USAGE ( .BOTH. , #39884 ) ;
#28508=ORIENTED_EDGE ( 'NONE', *, *, #25046, .F. ) ;
#28596=CIRCLE ( 'NONE', #36245, 0.3100393700787401619 ) ;
#28627=CARTESIAN_POINT ( 'NONE',  ( -0.3070839322311867403, -0.04408052624949946457, -1.037775876589189794 ) ) ;
#28641=ORIENTED_EDGE ( 'NONE', *, *, #17160, .F. ) ;
#28679=( LENGTH_UNIT ( ) NAMED_UNIT ( * ) SI_UNIT ( $, .METRE. ) ) ;
#28779=CARTESIAN_POINT ( 'NONE',  ( 0.000000000000000000, 0.000000000000000000, 1.181102362204724310 ) ) ;
#28794=DIRECTION ( 'NONE',  ( 0.000000000000000000, 0.000000000000000000, -1.000000000000000000 ) ) ;
#28865=CARTESIAN_POINT ( 'NONE',  ( -0.2984316586355673651, -0.08457185433607496139, -1.020769733662646672 ) ) ;
#28986=PLANE ( 'NONE',  #34903 ) ;
#29005=CARTESIAN_POINT ( 'NONE',  ( -0.2983856243743982506, 0.08472875797579371149, -1.020674147059416503 ) ) ;
#29112=CARTESIAN_POINT ( 'NONE',  ( -0.2802233088437621755, -0.1328339237432896724, -0.7736657976934293579 ) ) ;
#29118=LINE ( 'NONE', #14695, #12865 ) ;
#29239=DIRECTION ( 'NONE',  ( -1.000000000000000000, 0.000000000000000000, -0.000000000000000000 ) ) ;
#29259=CARTESIAN_POINT ( 'NONE',  ( -0.2896382684968236143, 0.1109106728611159998, -1.001724715795912601 ) ) ;
#29289=DIRECTION ( 'NONE',  ( 1.000000000000000000, -0.000000000000000000, -0.000000000000000000 ) ) ;
#29466=CARTESIAN_POINT ( 'NONE',  ( 0.2395294000716133853, 0.1968503937007874127, -0.4921259842519684069 ) ) ;
#29491=CARTESIAN_POINT ( 'NONE',  ( -0.2896200801440089734, 0.1109568837733818092, -0.7502863005648467976 ) ) ;
#29703=ADVANCED_FACE ( 'NONE', ( #30453 ), #37359, .T. ) ;
#29705=FACE_OUTER_BOUND ( 'NONE', #33177, .T. ) ;
#29756=CYLINDRICAL_SURFACE ( 'NONE', #32131, 0.3100393700787401619 ) ;
#29801=ADVANCED_FACE ( 'NONE', ( #15110 ), #29756, .T. ) ;
#29837=VERTEX_POINT ( 'NONE', #685 ) ;
#29839=CARTESIAN_POINT ( 'NONE',  ( -0.3100393700787401619, -0.01129866958151448837, 0.7086614173228350522 ) ) ;
#29983=AXIS2_PLACEMENT_3D ( 'NONE', #16951, #43034, #9998 ) ;
#29984=CARTESIAN_POINT ( 'NONE',  ( -0.2896382684968237808, 0.1109106728611156251, 0.7502437881410954912 ) ) ;
#30269=ORIENTED_EDGE ( 'NONE', *, *, #42114, .F. ) ;
#30363=EDGE_CURVE ( 'NONE', #18878, #27285, #11693, .T. ) ;
#30445=CARTESIAN_POINT ( 'NONE',  ( -0.2983856243743983061, 0.08472875797579337842, 0.7312943568775917003 ) ) ;
#30453=FACE_OUTER_BOUND ( 'NONE', #33004, .T. ) ;
#30507=DIRECTION ( 'NONE',  ( 0.000000000000000000, 0.000000000000000000, 1.000000000000000000 ) ) ;
#30660=DIRECTION ( 'NONE',  ( 1.000000000000000000, -0.000000000000000000, -0.000000000000000000 ) ) ;
#30673=EDGE_CURVE ( 'NONE', #18878, #1893, #16004, .T. ) ;
#30825=ORIENTED_EDGE ( 'NONE', *, *, #41668, .T. ) ;
#30996=CARTESIAN_POINT ( 'NONE',  ( -0.2664910633248679939, -0.1585270522231945201, 0.9306302837667671524 ) ) ;
#31027=EDGE_CURVE ( 'NONE', #1651, #18878, #37520, .T. ) ;
#31085=DIRECTION ( 'NONE',  ( 1.000000000000000000, -0.000000000000000000, -0.000000000000000000 ) ) ;
#31226=CARTESIAN_POINT ( 'NONE',  ( -0.3010365421720465617, -0.07487990393731483452, 1.026013379696918859 ) ) ;
#31318=EDGE_LOOP ( 'NONE', ( #7184, #44614, #9829, #26752 ) ) ;
#31966=CARTESIAN_POINT ( 'NONE',  ( -0.2624241468390501320, -0.1651049555683126169, -0.8482729357033111928 ) ) ;
#32113=DIRECTION ( 'NONE',  ( 1.000000000000000000, 0.000000000000000000, 0.000000000000000000 ) ) ;
#32125=DIRECTION ( 'NONE',  ( 0.000000000000000000, -1.000000000000000000, 0.000000000000000000 ) ) ;
#32131=AXIS2_PLACEMENT_3D ( 'NONE', #44303, #26129, #1402 ) ;
#32167=EDGE_CURVE ( 'NONE', #23773, #18452, #25333, .T. ) ;
#32202=CARTESIAN_POINT ( 'NONE',  ( -0.3100393700787401063, -0.01129866958151416051, -1.043307086614172485 ) ) ;
#32228=CARTESIAN_POINT ( 'NONE',  ( -0.3100393700787401619, 0.000000000000000000, -1.181102362204724310 ) ) ;
#32366=CARTESIAN_POINT ( 'NONE',  ( 0.000000000000000000, 0.000000000000000000, 0.4921259842519685179 ) ) ;
#32454=CARTESIAN_POINT ( 'NONE',  ( -0.2665235116888311495, -0.1584712422872020798, -0.9307722131276843225 ) ) ;
#32463=ADVANCED_FACE ( 'NONE', ( #44520 ), #19128, .T. ) ;
#32571=FACE_OUTER_BOUND ( 'NONE', #18522, .T. ) ;
#32586=CARTESIAN_POINT ( 'NONE',  ( -0.2833714012347086642, 0.1260629598319809863, -0.7654422454633916795 ) ) ;
#32610=ORIENTED_EDGE ( 'NONE', *, *, #45214, .F. ) ;
#32632=VECTOR ( 'NONE', #41028, 39.37007874015748143 ) ;
#32652=DIRECTION ( 'NONE',  ( 0.000000000000000000, 0.000000000000000000, 1.000000000000000000 ) ) ;
#32685=CARTESIAN_POINT ( 'NONE',  ( -0.2801779484932497843, -0.1329283866310993489, -0.9781771623220059109 ) ) ;
#32711=VERTEX_POINT ( 'NONE', #43048 ) ;
#32740=FILL_AREA_STYLE_COLOUR ( '', #10039 ) ;
#33004=EDGE_LOOP ( 'NONE', ( #42081, #26311, #40418 ) ) ;
#33046=CIRCLE ( 'NONE', #29983, 0.3100393700787401619 ) ;
#33088=CARTESIAN_POINT ( 'NONE',  ( -0.2610236670165032025, 0.1673052798952541498, 0.8873490049157347626 ) ) ;
#33162=ORIENTED_EDGE ( 'NONE', *, *, #18298, .F. ) ;
#33177=EDGE_LOOP ( 'NONE', ( #4082, #3333, #18991, #41529 ) ) ;
#33294=CARTESIAN_POINT ( 'NONE',  ( -0.2926984831716178959, 0.1026671379286199781, -1.008549658312261510 ) ) ;
#33511=VERTEX_POINT ( 'NONE', #1442 ) ;
#33525=CARTESIAN_POINT ( 'NONE',  ( -0.3100393700787402174, 0.01114154383210021713, -0.7086614173228347191 ) ) ;
#33557=CARTESIAN_POINT ( 'NONE',  ( -0.3100393700787402174, 0.01114154383210022407, 1.043307086614173151 ) ) ;
#33570=EDGE_LOOP ( 'NONE', ( #38193, #18754, #24707, #17388 ) ) ;
#33784=EDGE_LOOP ( 'NONE', ( #27818, #22253, #19889, #38602 ) ) ;
#33792=CARTESIAN_POINT ( 'NONE',  ( 0.000000000000000000, 0.000000000000000000, 1.181102362204724310 ) ) ;
#33884=CARTESIAN_POINT ( 'NONE',  ( 0.2395294000716133853, 3.423225304703229610E-16, -0.7086614173228351632 ) ) ;
#33889=VERTEX_POINT ( 'NONE', #29466 ) ;
#33920=PRODUCT_DEFINITION ( 'UNKNOWN', '', #46138, #39368 ) ;
#34071=AXIS2_PLACEMENT_3D ( 'NONE', #3264, #39204, #9995 ) ;
#34257=B_SPLINE_CURVE_WITH_KNOTS ( 'NONE', 3,
 ( #18761, #29839, #11359, #44382, #11593, #26217, #8208, #10897, #22600, #43932, #4359, #40088, #23554, #20176, #5565, #26690, #4845, #45334, #15670, #41959, #12779, #8930, #30996, #41242, #13009, #27415, #9166, #45559, #27173, #1728, #31226, #38395, #24028, #19709, #5087, #34350, #9410, #37692 ),
 .UNSPECIFIED., .F., .F.,
 ( 4, 2, 2, 2, 2, 2, 2, 2, 2, 2, 2, 2, 2, 2, 2, 2, 2, 2, 4 ),
 ( 0.000000000000000000, 0.0008476847199669325589, 0.001695369439933865118, 0.002543054159900797785, 0.003390738879867730236, 0.004238423599834662686, 0.005086108319801595570, 0.005933793039768528454, 0.006781477759735462206, 0.007205320119718934720, 0.007629162479702406366, 0.008476847199669360067, 0.009324531919636313768, 0.01017221663960326747, 0.01101990135957022117, 0.01186758607953717487, 0.01229142843952065259, 0.01271527079950412857, 0.01356295551947108401 ),
 .UNSPECIFIED. ) ;
#34341=DIRECTION ( 'NONE',  ( 1.000000000000000000, -0.000000000000000000, -0.000000000000000000 ) ) ;
#34350=CARTESIAN_POINT ( 'NONE',  ( -0.3094378032379022647, -0.02221465895966917917, 1.042200290985264344 ) ) ;
#34463=DIRECTION ( 'NONE',  ( -1.000000000000000000, 0.000000000000000000, 0.000000000000000000 ) ) ;
#34475=DIRECTION ( 'NONE',  ( 0.000000000000000000, 0.000000000000000000, -1.000000000000000000 ) ) ;
#34721=LINE ( 'NONE', #4985, #40816 ) ;
#34729=CARTESIAN_POINT ( 'NONE',  ( 0.2395294000716134131, 0.000000000000000000, 0.8759842519685039353 ) ) ;
#34826=CARTESIAN_POINT ( 'NONE',  ( -0.3100393700787401619, -2.714815113292586694E-26, -0.7086614173228351632 ) ) ;
#34903=AXIS2_PLACEMENT_3D ( 'NONE', #46666, #7380, #29239 ) ;
#34970=CARTESIAN_POINT ( 'NONE',  ( -0.3094147346904633777, 0.02254976514608433499, 0.7098108543537183790 ) ) ;
#35327=CARTESIAN_POINT ( 'NONE',  ( -0.2896766839110012648, -0.1108097609387615201, -0.7501563460709702591 ) ) ;
#35559=CARTESIAN_POINT ( 'NONE',  ( -0.3100393700787403284, -0.01116717051762143413, -0.7086614173228348301 ) ) ;
#35658=VECTOR ( 'NONE', #7286, 39.37007874015748143 ) ;
#36097=FACE_OUTER_BOUND ( 'NONE', #16479, .T. ) ;
#36225=ADVANCED_FACE ( 'NONE', ( #41973 ), #9181, .T. ) ;
#36245=AXIS2_PLACEMENT_3D ( 'NONE', #28779, #6209, #20838 ) ;
#36297=ORIENTED_EDGE ( 'NONE', *, *, #7261, .T. ) ;
#36332=ORIENTED_EDGE ( 'NONE', *, *, #13087, .F. ) ;
#36391=FACE_OUTER_BOUND ( 'NONE', #33570, .T. ) ;
#36548=DIRECTION ( 'NONE',  ( -0.000000000000000000, -0.000000000000000000, -1.000000000000000000 ) ) ;
#36554=CYLINDRICAL_SURFACE ( 'NONE', #9246, 0.1673228346456687721 ) ;
#36628=CARTESIAN_POINT ( 'NONE',  ( -0.3053406547161472417, 0.05476901150469701274, -0.7174944170560512147 ) ) ;
#36658=CARTESIAN_POINT ( 'NONE',  ( -0.3070711847658871285, 0.04416910270118645093, 1.037751739429055409 ) ) ;
#36824=MECHANICAL_DESIGN_GEOMETRIC_PRESENTATION_REPRESENTATION('',(#7733),#23783);
#36860=CARTESIAN_POINT ( 'NONE',  ( -0.2741498948998220553, 0.1449524278970012459, -0.9602547136744080669 ) ) ;
#36895=CARTESIAN_POINT ( 'NONE',  ( -0.2664436179446795228, 0.1586070934160168089, 0.8215608667368892171 ) ) ;
#37067=CYLINDRICAL_SURFACE ( 'NONE', #8359, 0.1673228346456687721 ) ;
#37121=CARTESIAN_POINT ( 'NONE',  ( -0.2610014219173109051, 0.1673399808196281979, 0.8651424297200356328 ) ) ;
#37211=ORIENTED_EDGE ( 'NONE', *, *, #40264, .F. ) ;
#37221=ADVANCED_FACE ( 'NONE', ( #3813, #21077 ), #7412, .F. ) ;
#37242=VERTEX_POINT ( 'NONE', #18432 ) ;
#37316=CARTESIAN_POINT ( 'NONE',  ( -0.2665307357296560209, 0.1584585643853064219, -0.8211671128013016130 ) ) ;
#37359=PLANE ( 'NONE',  #42787 ) ;
#37414=ORIENTED_EDGE ( 'NONE', *, *, #40264, .T. ) ;
#37434=CARTESIAN_POINT ( 'NONE',  ( 0.2395294000716133853, -0.1968503937007874127, -0.4921259842519685179 ) ) ;
#37509=CARTESIAN_POINT ( 'NONE',  ( 0.000000000000000000, 0.000000000000000000, 0.4921259842519685179 ) ) ;
#37520=CIRCLE ( 'NONE', #9239, 0.3100393700787401619 ) ;
#37554=EDGE_CURVE ( 'NONE', #1893, #2328, #21082, .T. ) ;
#37561=CARTESIAN_POINT ( 'NONE',  ( -0.3053042314538800817, 0.05494681823601590964, -1.034402892550617459 ) ) ;
#37692=CARTESIAN_POINT ( 'NONE',  ( -0.3100393700787401619, -2.714815113292586694E-26, 1.043307086614172707 ) ) ;
#37716=ADVANCED_FACE ( 'NONE', ( #3106 ), #39752, .F. ) ;
#37935=VERTEX_POINT ( 'NONE', #26839 ) ;
#37994=APPLICATION_CONTEXT ( 'automotive_design' ) ;
#38077=CARTESIAN_POINT ( 'NONE',  ( -0.3100393700787402174, 0.01127274112884909044, 0.7086614173228353852 ) ) ;
#38193=ORIENTED_EDGE ( 'NONE', *, *, #47187, .T. ) ;
#38262=CARTESIAN_POINT ( 'NONE',  ( 0.3100393700787401619, 3.796887221765908018E-17, 0.4921259842519685179 ) ) ;
#38357=ADVANCED_FACE ( 'NONE', ( #32571 ), #28986, .T. ) ;
#38358=EDGE_CURVE ( 'NONE', #18450, #1893, #18056, .T. ) ;
#38395=CARTESIAN_POINT ( 'NONE',  ( -0.3042596054108611114, -0.05980719604265498368, 1.032348353801579410 ) ) ;
#38448=ORIENTED_EDGE ( 'NONE', *, *, #8498, .T. ) ;
#38465=PRODUCT ( 'Pivot Shaft', 'Pivot Shaft', '', ( #15200 ) ) ;
#38551=CARTESIAN_POINT ( 'NONE',  ( 0.3100393700787401619, 3.796887221765908018E-17, -0.4921259842519685179 ) ) ;
#38602=ORIENTED_EDGE ( 'NONE', *, *, #20592, .T. ) ;
#38772=EDGE_LOOP ( 'NONE', ( #9577, #23478 ) ) ;
#39178=SURFACE_STYLE_FILL_AREA ( #24811 ) ;
#39204=DIRECTION ( 'NONE',  ( 0.000000000000000000, 0.000000000000000000, -1.000000000000000000 ) ) ;
#39368=PRODUCT_DEFINITION_CONTEXT ( 'detailed design', #46508, 'design' ) ;
#39620=EDGE_LOOP ( 'NONE', ( #37414, #40405, #22539, #27463 ) ) ;
#39675=ORIENTED_EDGE ( 'NONE', *, *, #31027, .F. ) ;
#39752=CYLINDRICAL_SURFACE ( 'NONE', #42454, 0.1673228346456687721 ) ;
#39824=CARTESIAN_POINT ( 'NONE',  ( -0.2664910633248679939, -0.1585270522231942703, -0.8213382201702412733 ) ) ;
#39834=UNCERTAINTY_MEASURE_WITH_UNIT (LENGTH_MEASURE( 1.000000000000000082E-05 ), #9122, 'distance_accuracy_value', 'NONE') ;
#39884=SURFACE_SIDE_STYLE ('',( #39178 ) ) ;
#39961=CARTESIAN_POINT ( 'NONE',  ( -0.2927386332256519674, 0.1025512834716172661, -0.7433308942907063122 ) ) ;
#40088=CARTESIAN_POINT ( 'NONE',  ( -0.2741503469832764495, -0.1449524958156370724, 0.7917101702132945951 ) ) ;
#40222=CARTESIAN_POINT ( 'NONE',  ( 0.2395294000716133853, -0.1968503937007874127, -0.4921259842519685179 ) ) ;
#40264=EDGE_CURVE ( 'NONE', #37935, #29837, #21432, .T. ) ;
#40374=DIRECTION ( 'NONE',  ( 0.000000000000000000, 0.000000000000000000, 1.000000000000000000 ) ) ;
#40405=ORIENTED_EDGE ( 'NONE', *, *, #22168, .F. ) ;
#40418=ORIENTED_EDGE ( 'NONE', *, *, #24783, .F. ) ;
#40429=CARTESIAN_POINT ( 'NONE',  ( -0.2610014219173106831, 0.1673399808196284755, -0.8868260742169717936 ) ) ;
#40800=CYLINDRICAL_SURFACE ( 'NONE', #7264, 0.1673228346456687721 ) ;
#40816=VECTOR ( 'NONE', #30660, 39.37007874015748143 ) ;
#40878=PLANE ( 'NONE',  #44331 ) ;
#40883=AXIS2_PLACEMENT_3D ( 'NONE', #17521, #20641, #6494 ) ;
#40894=CARTESIAN_POINT ( 'NONE',  ( -0.2713383277233170632, 0.1500775187160215962, -0.8012127751235805784 ) ) ;
#41028=DIRECTION ( 'NONE',  ( 1.000000000000000000, -0.000000000000000000, -0.000000000000000000 ) ) ;
#41189=ORIENTED_EDGE ( 'NONE', *, *, #13221, .T. ) ;
#41242=CARTESIAN_POINT ( 'NONE',  ( -0.2713569170882992876, -0.1500457819031514040, 0.9508393013034962538 ) ) ;
#41396=CARTESIAN_POINT ( 'NONE',  ( -0.3010001048904012988, 0.07502508536398720673, 0.7260280747557159575 ) ) ;
#41429=CARTESIAN_POINT ( 'NONE',  ( -0.3100393700787401619, 0.000000000000000000, 1.181102362204724310 ) ) ;
#41529=ORIENTED_EDGE ( 'NONE', *, *, #30673, .T. ) ;
#41575=EDGE_CURVE ( 'NONE', #47237, #23773, #23311, .T. ) ;
#41585=DIRECTION ( 'NONE',  ( -0.000000000000000000, -0.000000000000000000, 1.000000000000000000 ) ) ;
#41592=LINE ( 'NONE', #23663, #47107 ) ;
#41668=EDGE_CURVE ( 'NONE', #18452, #23773, #14140, .T. ) ;
#41865=DIRECTION ( 'NONE',  ( 1.000000000000000000, -0.000000000000000000, -0.000000000000000000 ) ) ;
#41959=CARTESIAN_POINT ( 'NONE',  ( -0.2618967166504349020, -0.1659366058165111513, 0.8981965965474308922 ) ) ;
#41973=FACE_OUTER_BOUND ( 'NONE', #47186, .T. ) ;
#42079=LINE ( 'NONE', #4961, #23659 ) ;
#42081=ORIENTED_EDGE ( 'NONE', *, *, #37554, .F. ) ;
#42112=CARTESIAN_POINT ( 'NONE',  ( -0.3053042314538801927, 0.05494681823601579862, 0.7175656113863903007 ) ) ;
#42114=EDGE_CURVE ( 'NONE', #16713, #29837, #22574, .T. ) ;
#42150=ORIENTED_EDGE ( 'NONE', *, *, #24787, .T. ) ;
#42155=( NAMED_UNIT ( * ) PLANE_ANGLE_UNIT ( ) SI_UNIT ( $, .RADIAN. ) ) ;
#42341=AXIS2_PLACEMENT_3D ( 'NONE', #32366, #17715, #32113 ) ;
#42416=VERTEX_POINT ( 'NONE', #45451 ) ;
#42454=AXIS2_PLACEMENT_3D ( 'NONE', #6942, #29289, #28794 ) ;
#42459=DIRECTION ( 'NONE',  ( 0.000000000000000000, 0.000000000000000000, -1.000000000000000000 ) ) ;
#42727=LINE ( 'NONE', #20246, #834 ) ;
#42787=AXIS2_PLACEMENT_3D ( 'NONE', #11506, #45252, #12472 ) ;
#42943=CARTESIAN_POINT ( 'NONE',  ( -0.2644738720849209024, -0.1618167320693821298, -0.8319978239451156776 ) ) ;
#43034=DIRECTION ( 'NONE',  ( 0.000000000000000000, 0.000000000000000000, -1.000000000000000000 ) ) ;
#43048=CARTESIAN_POINT ( 'NONE',  ( 0.2395294000716134131, 2.049113738730802390E-17, 1.043307086614172929 ) ) ;
#43136=DIRECTION ( 'NONE',  ( 1.000000000000000000, -0.000000000000000000, -0.000000000000000000 ) ) ;
#43163=EDGE_CURVE ( 'NONE', #37935, #16713, #5781, .T. ) ;
#43232=CARTESIAN_POINT ( 'NONE',  ( 0.2395294000716133853, -0.1968503937007874127, -1.181102362204724310 ) ) ;
#43665=CARTESIAN_POINT ( 'NONE',  ( -0.2834275672170630811, -0.1259372798753285727, -0.7652988122780589597 ) ) ;
#43677=AXIS2_PLACEMENT_3D ( 'NONE', #13549, #31085, #20959 ) ;
#43712=DIRECTION ( 'NONE',  ( 0.000000000000000000, 1.000000000000000000, 0.000000000000000000 ) ) ;
#43722=FACE_OUTER_BOUND ( 'NONE', #8332, .T. ) ;
#43762=EDGE_CURVE ( 'NONE', #33511, #32711, #44866, .T. ) ;
#43770=EDGE_LOOP ( 'NONE', ( #39675, #8721, #13509, #1391, #30269, #23426, #36332, #28508, #9328, #5860, #3244, #19094 ) ) ;
#43813=( GEOMETRIC_REPRESENTATION_CONTEXT ( 3 ) GLOBAL_UNCERTAINTY_ASSIGNED_CONTEXT ( ( #39834 ) ) GLOBAL_UNIT_ASSIGNED_CONTEXT ( ( #9122, #42155, #23985 ) ) REPRESENTATION_CONTEXT ( 'NONE', 'WORKASPACE' ) ) ;
#43847=ORIENTED_EDGE ( 'NONE', *, *, #46510, .T. ) ;
#43932=CARTESIAN_POINT ( 'NONE',  ( -0.2833820772873879568, -0.1260390447071885467, 0.7654149962237527527 ) ) ;
#44035=CARTESIAN_POINT ( 'NONE',  ( -0.2741699206993515880, 0.1449164722121961124, -0.7916449048462085303 ) ) ;
#44044=ORIENTED_EDGE ( 'NONE', *, *, #45214, .T. ) ;
#44303=CARTESIAN_POINT ( 'NONE',  ( 0.000000000000000000, 0.000000000000000000, 1.181102362204724310 ) ) ;
#44331=AXIS2_PLACEMENT_3D ( 'NONE', #11935, #22937, #4707 ) ;
#44382=CARTESIAN_POINT ( 'NONE',  ( -0.3070839322311865738, -0.04408052624949979070, 0.7141926273478177434 ) ) ;
#44520=FACE_OUTER_BOUND ( 'NONE', #43770, .T. ) ;
#44614=ORIENTED_EDGE ( 'NONE', *, *, #41575, .T. ) ;
#44630=CARTESIAN_POINT ( 'NONE',  ( 0.2395294000716133853, 3.218313930830148909E-16, -0.8759842519685039353 ) ) ;
#44866=LINE ( 'NONE', #26701, #32632 ) ;
#44979=ADVANCED_BREP_SHAPE_REPRESENTATION ( 'Pivot Shaft', ( #20411, #20860 ), #43813 ) ;
#44999=CARTESIAN_POINT ( 'NONE',  ( -0.3070313825494069282, 0.04447134000132128145, 0.7142919828228455614 ) ) ;
#45142=VECTOR ( 'NONE', #41585, 39.37007874015748143 ) ;
#45214=EDGE_CURVE ( 'NONE', #19863, #15025, #33046, .T. ) ;
#45252=DIRECTION ( 'NONE',  ( 0.000000000000000000, -0.000000000000000000, 1.000000000000000000 ) ) ;
#45273=LINE ( 'NONE', #41429, #16466 ) ;
#45334=CARTESIAN_POINT ( 'NONE',  ( -0.2610081115717080569, -0.1673295453843250680, 0.8813693982766842572 ) ) ;
#45451=CARTESIAN_POINT ( 'NONE',  ( -0.3100393700787401619, 3.218313930830148909E-16, -1.043307086614172707 ) ) ;
#45478=ORIENTED_EDGE ( 'NONE', *, *, #43163, .T. ) ;
#45559=CARTESIAN_POINT ( 'NONE',  ( -0.2896766839110013758, -0.1108097609387616589, 1.001812157866037722 ) ) ;
#45870=EDGE_CURVE ( 'NONE', #15025, #37935, #42727, .T. ) ;
#46093=ORIENTED_EDGE ( 'NONE', *, *, #11537, .F. ) ;
#46138=PRODUCT_DEFINITION_FORMATION_WITH_SPECIFIED_SOURCE ( 'ANY', '', #38465, .NOT_KNOWN. ) ;
#46508=APPLICATION_CONTEXT ( 'automotive_design' ) ;
#46510=EDGE_CURVE ( 'NONE', #33889, #19863, #25406, .T. ) ;
#46551=CARTESIAN_POINT ( 'NONE',  ( -0.2984771744461587328, -0.08441368980803262700, -0.7311049032655659863 ) ) ;
#46666=CARTESIAN_POINT ( 'NONE',  ( 0.000000000000000000, 0.000000000000000000, -1.181102362204724310 ) ) ;
#46788=CARTESIAN_POINT ( 'NONE',  ( -0.2713569170882992876, -0.1500457819031512374, -0.8011292026335117278 ) ) ;
#47031=CARTESIAN_POINT ( 'NONE',  ( -0.3076751137723114371, -0.03860885780051061950, -0.7130813053422531134 ) ) ;
#47084=DIRECTION ( 'NONE',  ( 1.000000000000000000, -0.000000000000000000, -0.000000000000000000 ) ) ;
#47107=VECTOR ( 'NONE', #8798, 39.37007874015748143 ) ;
#47186=EDGE_LOOP ( 'NONE', ( #43847, #44044, #17576 ) ) ;
#47187=EDGE_CURVE ( 'NONE', #19692, #33511, #34257, .T. ) ;
#47237=VERTEX_POINT ( 'NONE', #34826 ) ;
#47275=CARTESIAN_POINT ( 'NONE',  ( -0.2611872605799127056, -0.1670510767787601047, -0.8649260808424121816 ) ) ;
#47336=PRESENTATION_STYLE_ASSIGNMENT (( #28432 ) ) ;
#47411=CARTESIAN_POINT ( 'NONE',  ( -0.3100393700787401619, -2.714815113292586694E-26, -0.7086614173228351632 ) ) ;
ENDSEC;
END-ISO-10303-21;
